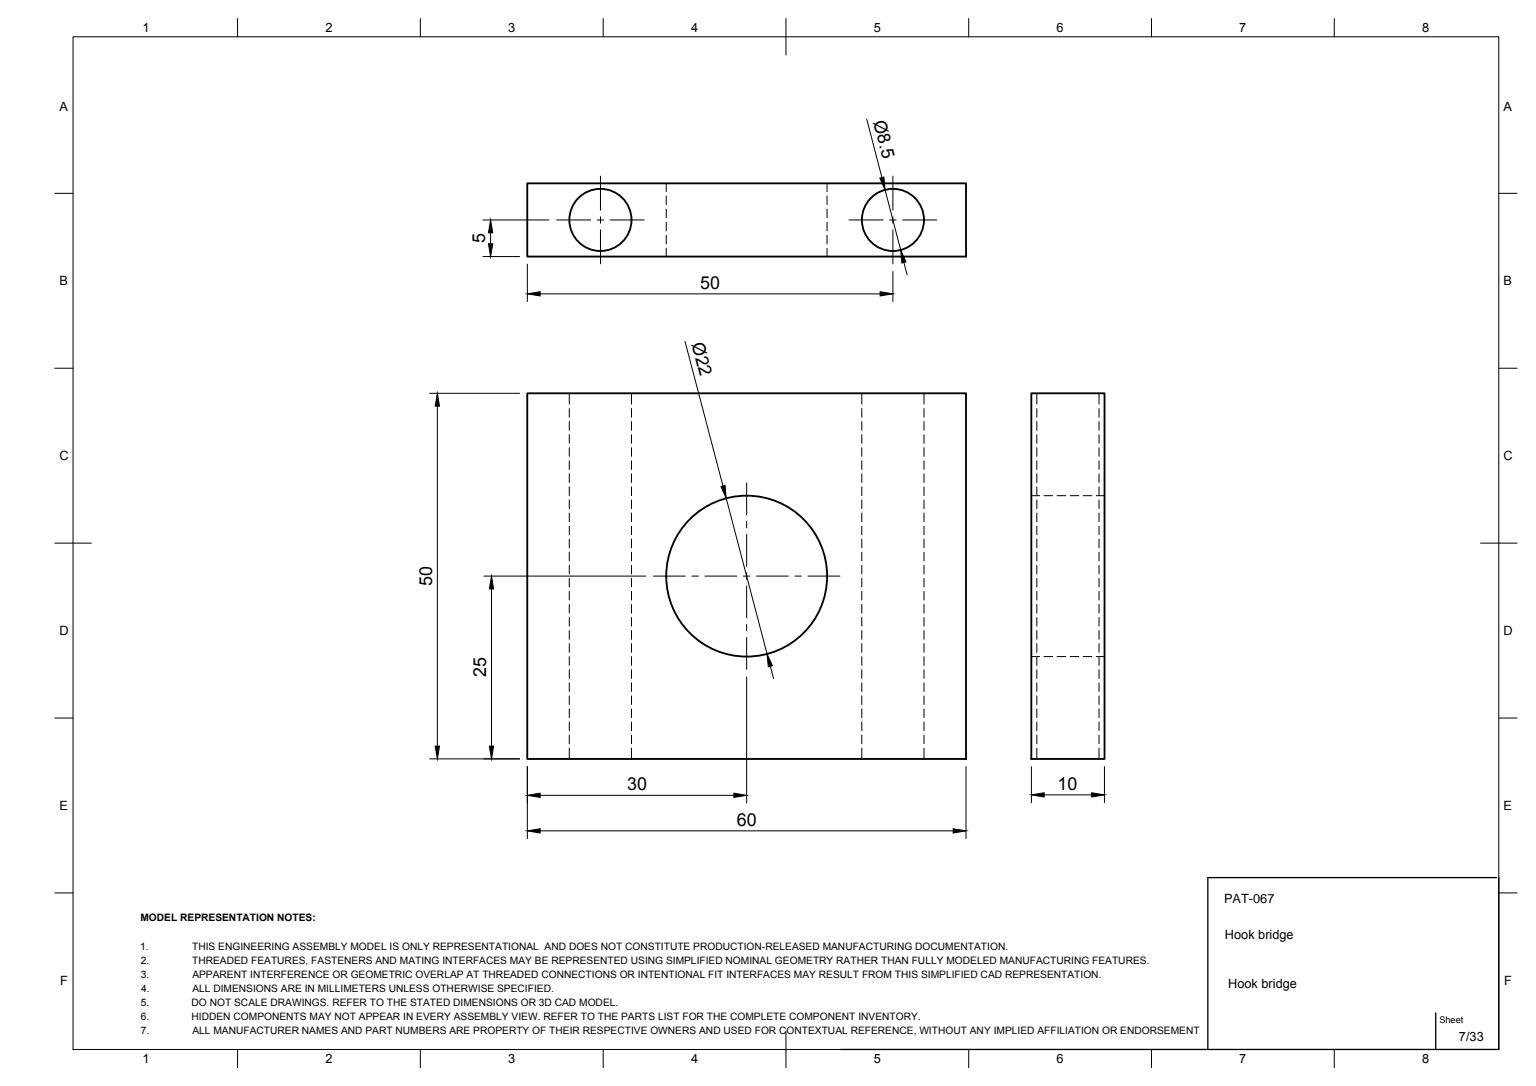
ISO-10303-21;
HEADER;
/* Generated by software containing ST-Developer
 * from STEP Tools, Inc. (www.steptools.com) 
 */

FILE_DESCRIPTION(
/* description */ ('Lifting hook block with sheave'),
/* implementation_level */ '2;1');

FILE_NAME(
/* name */ 'Hook bridge.step',
/* time_stamp */ '2026-10-28T03:23:54-07:00',
/* author */ (''),
/* organization */ (''),
/* preprocessor_version */ 'ST-DEVELOPER v20.2',
/* originating_system */ 'Autodesk Translation Framework v15.17.0.0',
/* authorisation */ '');

FILE_SCHEMA (('AUTOMOTIVE_DESIGN { 1 0 10303 214 3 1 1 }'));
ENDSEC;

DATA;
#10=MECHANICAL_DESIGN_GEOMETRIC_PRESENTATION_REPRESENTATION('',(#353),#9391);
#293=SHAPE_REPRESENTATION_RELATIONSHIP('SRR','None',#9524,#323);
#323=ADVANCED_BREP_SHAPE_REPRESENTATION('',(#391),#9359);
#353=STYLED_ITEM('',(#9773),#391);
#391=MANIFOLD_SOLID_BREP('Body1',#4889);
#506=LINE('',#7866,#794);
#507=LINE('',#7872,#795);
#508=LINE('',#7878,#796);
#509=LINE('',#7883,#797);
#510=LINE('',#7885,#798);
#511=LINE('',#7887,#799);
#512=LINE('',#7888,#800);
#513=LINE('',#7891,#801);
#514=LINE('',#7893,#802);
#515=LINE('',#7894,#803);
#516=LINE('',#7897,#804);
#517=LINE('',#7899,#805);
#518=LINE('',#7900,#806);
#519=LINE('',#7902,#807);
#520=LINE('',#7903,#808);
#794=VECTOR('',#6261,1.1);
#795=VECTOR('',#6268,0.425);
#796=VECTOR('',#6275,0.425);
#797=VECTOR('',#6280,1.);
#798=VECTOR('',#6281,1.);
#799=VECTOR('',#6282,1.);
#800=VECTOR('',#6283,1.);
#801=VECTOR('',#6286,1.);
#802=VECTOR('',#6287,1.);
#803=VECTOR('',#6288,1.);
#804=VECTOR('',#6291,1.);
#805=VECTOR('',#6292,1.);
#806=VECTOR('',#6293,1.);
#807=VECTOR('',#6296,1.);
#808=VECTOR('',#6297,1.);
#1026=CYLINDRICAL_SURFACE('',#5382,1.1);
#1027=CYLINDRICAL_SURFACE('',#5385,0.425);
#1028=CYLINDRICAL_SURFACE('',#5388,0.425);
#1135=FACE_BOUND('',#1593,.T.);
#1136=FACE_BOUND('',#1594,.T.);
#1137=FACE_BOUND('',#1597,.T.);
#1138=FACE_BOUND('',#1598,.T.);
#1139=FACE_BOUND('',#1601,.T.);
#1140=FACE_BOUND('',#1603,.T.);
#1272=FACE_OUTER_BOUND('',#1589,.T.);
#1273=FACE_OUTER_BOUND('',#1590,.T.);
#1274=FACE_OUTER_BOUND('',#1591,.T.);
#1275=FACE_OUTER_BOUND('',#1592,.T.);
#1276=FACE_OUTER_BOUND('',#1595,.T.);
#1277=FACE_OUTER_BOUND('',#1596,.T.);
#1278=FACE_OUTER_BOUND('',#1599,.T.);
#1279=FACE_OUTER_BOUND('',#1600,.T.);
#1280=FACE_OUTER_BOUND('',#1602,.T.);
#1589=EDGE_LOOP('',(#3530,#3531,#3532,#3533));
#1590=EDGE_LOOP('',(#3534,#3535,#3536,#3537));
#1591=EDGE_LOOP('',(#3538,#3539,#3540,#3541));
#1592=EDGE_LOOP('',(#3542,#3543,#3544,#3545));
#1593=EDGE_LOOP('',(#3546));
#1594=EDGE_LOOP('',(#3547));
#1595=EDGE_LOOP('',(#3548,#3549,#3550,#3551));
#1596=EDGE_LOOP('',(#3552,#3553,#3554,#3555));
#1597=EDGE_LOOP('',(#3556));
#1598=EDGE_LOOP('',(#3557));
#1599=EDGE_LOOP('',(#3558,#3559,#3560,#3561));
#1600=EDGE_LOOP('',(#3562,#3563,#3564,#3565));
#1601=EDGE_LOOP('',(#3566));
#1602=EDGE_LOOP('',(#3567,#3568,#3569,#3570));
#1603=EDGE_LOOP('',(#3571));
#1983=CIRCLE('',#5383,1.1);
#1984=CIRCLE('',#5384,1.1);
#1985=CIRCLE('',#5386,0.425);
#1986=CIRCLE('',#5387,0.425);
#1987=CIRCLE('',#5389,0.425);
#1988=CIRCLE('',#5390,0.425);
#2308=VERTEX_POINT('',#7863);
#2309=VERTEX_POINT('',#7865);
#2310=VERTEX_POINT('',#7869);
#2311=VERTEX_POINT('',#7871);
#2312=VERTEX_POINT('',#7875);
#2313=VERTEX_POINT('',#7877);
#2314=VERTEX_POINT('',#7881);
#2315=VERTEX_POINT('',#7882);
#2316=VERTEX_POINT('',#7884);
#2317=VERTEX_POINT('',#7886);
#2318=VERTEX_POINT('',#7890);
#2319=VERTEX_POINT('',#7892);
#2320=VERTEX_POINT('',#7896);
#2321=VERTEX_POINT('',#7898);
#2769=EDGE_CURVE('',#2308,#2308,#1983,.T.);
#2770=EDGE_CURVE('',#2308,#2309,#506,.T.);
#2771=EDGE_CURVE('',#2309,#2309,#1984,.T.);
#2772=EDGE_CURVE('',#2310,#2310,#1985,.T.);
#2773=EDGE_CURVE('',#2310,#2311,#507,.T.);
#2774=EDGE_CURVE('',#2311,#2311,#1986,.T.);
#2775=EDGE_CURVE('',#2312,#2312,#1987,.T.);
#2776=EDGE_CURVE('',#2312,#2313,#508,.T.);
#2777=EDGE_CURVE('',#2313,#2313,#1988,.T.);
#2778=EDGE_CURVE('',#2314,#2315,#509,.T.);
#2779=EDGE_CURVE('',#2315,#2316,#510,.T.);
#2780=EDGE_CURVE('',#2317,#2316,#511,.T.);
#2781=EDGE_CURVE('',#2314,#2317,#512,.T.);
#2782=EDGE_CURVE('',#2318,#2314,#513,.T.);
#2783=EDGE_CURVE('',#2319,#2317,#514,.T.);
#2784=EDGE_CURVE('',#2318,#2319,#515,.T.);
#2785=EDGE_CURVE('',#2320,#2318,#516,.T.);
#2786=EDGE_CURVE('',#2321,#2319,#517,.T.);
#2787=EDGE_CURVE('',#2320,#2321,#518,.T.);
#2788=EDGE_CURVE('',#2315,#2320,#519,.T.);
#2789=EDGE_CURVE('',#2316,#2321,#520,.T.);
#3530=ORIENTED_EDGE('',*,*,#2769,.F.);
#3531=ORIENTED_EDGE('',*,*,#2770,.T.);
#3532=ORIENTED_EDGE('',*,*,#2771,.F.);
#3533=ORIENTED_EDGE('',*,*,#2770,.F.);
#3534=ORIENTED_EDGE('',*,*,#2772,.F.);
#3535=ORIENTED_EDGE('',*,*,#2773,.T.);
#3536=ORIENTED_EDGE('',*,*,#2774,.F.);
#3537=ORIENTED_EDGE('',*,*,#2773,.F.);
#3538=ORIENTED_EDGE('',*,*,#2775,.F.);
#3539=ORIENTED_EDGE('',*,*,#2776,.T.);
#3540=ORIENTED_EDGE('',*,*,#2777,.F.);
#3541=ORIENTED_EDGE('',*,*,#2776,.F.);
#3542=ORIENTED_EDGE('',*,*,#2778,.T.);
#3543=ORIENTED_EDGE('',*,*,#2779,.T.);
#3544=ORIENTED_EDGE('',*,*,#2780,.F.);
#3545=ORIENTED_EDGE('',*,*,#2781,.F.);
#3546=ORIENTED_EDGE('',*,*,#2774,.T.);
#3547=ORIENTED_EDGE('',*,*,#2777,.T.);
#3548=ORIENTED_EDGE('',*,*,#2782,.T.);
#3549=ORIENTED_EDGE('',*,*,#2781,.T.);
#3550=ORIENTED_EDGE('',*,*,#2783,.F.);
#3551=ORIENTED_EDGE('',*,*,#2784,.F.);
#3552=ORIENTED_EDGE('',*,*,#2785,.T.);
#3553=ORIENTED_EDGE('',*,*,#2784,.T.);
#3554=ORIENTED_EDGE('',*,*,#2786,.F.);
#3555=ORIENTED_EDGE('',*,*,#2787,.F.);
#3556=ORIENTED_EDGE('',*,*,#2772,.T.);
#3557=ORIENTED_EDGE('',*,*,#2775,.T.);
#3558=ORIENTED_EDGE('',*,*,#2788,.T.);
#3559=ORIENTED_EDGE('',*,*,#2787,.T.);
#3560=ORIENTED_EDGE('',*,*,#2789,.F.);
#3561=ORIENTED_EDGE('',*,*,#2779,.F.);
#3562=ORIENTED_EDGE('',*,*,#2789,.T.);
#3563=ORIENTED_EDGE('',*,*,#2786,.T.);
#3564=ORIENTED_EDGE('',*,*,#2783,.T.);
#3565=ORIENTED_EDGE('',*,*,#2780,.T.);
#3566=ORIENTED_EDGE('',*,*,#2771,.T.);
#3567=ORIENTED_EDGE('',*,*,#2788,.F.);
#3568=ORIENTED_EDGE('',*,*,#2778,.F.);
#3569=ORIENTED_EDGE('',*,*,#2782,.F.);
#3570=ORIENTED_EDGE('',*,*,#2785,.F.);
#3571=ORIENTED_EDGE('',*,*,#2769,.T.);
#4476=PLANE('',#5391);
#4477=PLANE('',#5392);
#4478=PLANE('',#5393);
#4479=PLANE('',#5394);
#4480=PLANE('',#5395);
#4481=PLANE('',#5396);
#4648=ADVANCED_FACE('',(#1272),#1026,.F.);
#4649=ADVANCED_FACE('',(#1273),#1027,.F.);
#4650=ADVANCED_FACE('',(#1274),#1028,.F.);
#4651=ADVANCED_FACE('',(#1275,#1135,#1136),#4476,.T.);
#4652=ADVANCED_FACE('',(#1276),#4477,.T.);
#4653=ADVANCED_FACE('',(#1277,#1137,#1138),#4478,.T.);
#4654=ADVANCED_FACE('',(#1278),#4479,.T.);
#4655=ADVANCED_FACE('',(#1279,#1139),#4480,.T.);
#4656=ADVANCED_FACE('',(#1280,#1140),#4481,.F.);
#4889=CLOSED_SHELL('',(#4648,#4649,#4650,#4651,#4652,#4653,#4654,#4655,
#4656));
#5381=AXIS2_PLACEMENT_3D('',#7861,#6255,#6256);
#5382=AXIS2_PLACEMENT_3D('',#7862,#6257,#6258);
#5383=AXIS2_PLACEMENT_3D('',#7864,#6259,#6260);
#5384=AXIS2_PLACEMENT_3D('',#7867,#6262,#6263);
#5385=AXIS2_PLACEMENT_3D('',#7868,#6264,#6265);
#5386=AXIS2_PLACEMENT_3D('',#7870,#6266,#6267);
#5387=AXIS2_PLACEMENT_3D('',#7873,#6269,#6270);
#5388=AXIS2_PLACEMENT_3D('',#7874,#6271,#6272);
#5389=AXIS2_PLACEMENT_3D('',#7876,#6273,#6274);
#5390=AXIS2_PLACEMENT_3D('',#7879,#6276,#6277);
#5391=AXIS2_PLACEMENT_3D('',#7880,#6278,#6279);
#5392=AXIS2_PLACEMENT_3D('',#7889,#6284,#6285);
#5393=AXIS2_PLACEMENT_3D('',#7895,#6289,#6290);
#5394=AXIS2_PLACEMENT_3D('',#7901,#6294,#6295);
#5395=AXIS2_PLACEMENT_3D('',#7904,#6298,#6299);
#5396=AXIS2_PLACEMENT_3D('',#7905,#6300,#6301);
#6255=DIRECTION('axis',(0.,0.,1.));
#6256=DIRECTION('refdir',(1.,0.,0.));
#6257=DIRECTION('center_axis',(0.,0.,1.));
#6258=DIRECTION('ref_axis',(1.,0.,0.));
#6259=DIRECTION('center_axis',(0.,0.,1.));
#6260=DIRECTION('ref_axis',(1.,0.,0.));
#6261=DIRECTION('',(0.,0.,1.));
#6262=DIRECTION('center_axis',(0.,0.,-1.));
#6263=DIRECTION('ref_axis',(1.,0.,0.));
#6264=DIRECTION('center_axis',(0.,1.,0.));
#6265=DIRECTION('ref_axis',(1.,0.,0.));
#6266=DIRECTION('center_axis',(0.,1.,0.));
#6267=DIRECTION('ref_axis',(1.,0.,0.));
#6268=DIRECTION('',(0.,1.,0.));
#6269=DIRECTION('center_axis',(0.,-1.,0.));
#6270=DIRECTION('ref_axis',(1.,0.,0.));
#6271=DIRECTION('center_axis',(0.,1.,0.));
#6272=DIRECTION('ref_axis',(1.,0.,0.));
#6273=DIRECTION('center_axis',(0.,1.,0.));
#6274=DIRECTION('ref_axis',(1.,0.,0.));
#6275=DIRECTION('',(0.,1.,0.));
#6276=DIRECTION('center_axis',(0.,-1.,0.));
#6277=DIRECTION('ref_axis',(1.,0.,0.));
#6278=DIRECTION('center_axis',(0.,1.,0.));
#6279=DIRECTION('ref_axis',(-1.,0.,0.));
#6280=DIRECTION('',(-1.,0.,0.));
#6281=DIRECTION('',(0.,0.,1.));
#6282=DIRECTION('',(-1.,0.,0.));
#6283=DIRECTION('',(0.,0.,1.));
#6284=DIRECTION('center_axis',(1.,0.,0.));
#6285=DIRECTION('ref_axis',(0.,1.,0.));
#6286=DIRECTION('',(0.,1.,0.));
#6287=DIRECTION('',(0.,1.,0.));
#6288=DIRECTION('',(0.,0.,1.));
#6289=DIRECTION('center_axis',(0.,-1.,0.));
#6290=DIRECTION('ref_axis',(1.,0.,0.));
#6291=DIRECTION('',(1.,0.,0.));
#6292=DIRECTION('',(1.,0.,0.));
#6293=DIRECTION('',(0.,0.,1.));
#6294=DIRECTION('center_axis',(-1.,0.,0.));
#6295=DIRECTION('ref_axis',(0.,-1.,0.));
#6296=DIRECTION('',(0.,-1.,0.));
#6297=DIRECTION('',(0.,-1.,0.));
#6298=DIRECTION('center_axis',(0.,0.,1.));
#6299=DIRECTION('ref_axis',(1.,0.,0.));
#6300=DIRECTION('center_axis',(0.,0.,1.));
#6301=DIRECTION('ref_axis',(1.,0.,0.));
#7861=CARTESIAN_POINT('',(0.,0.,0.));
#7862=CARTESIAN_POINT('Origin',(0.,0.,4.4));
#7863=CARTESIAN_POINT('',(-1.1,-1.34711147906209E-16,4.5));
#7864=CARTESIAN_POINT('Origin',(0.,0.,4.5));
#7865=CARTESIAN_POINT('',(-1.1,1.34711147906209E-16,5.5));
#7866=CARTESIAN_POINT('',(-1.1,-1.34711147906209E-16,4.4));
#7867=CARTESIAN_POINT('Origin',(0.,0.,5.5));
#7868=CARTESIAN_POINT('Origin',(-2.,-2.6,5.));
#7869=CARTESIAN_POINT('',(-2.425,-2.5,5.));
#7870=CARTESIAN_POINT('Origin',(-2.,-2.5,5.));
#7871=CARTESIAN_POINT('',(-2.425,2.5,5.));
#7872=CARTESIAN_POINT('',(-2.425,-2.6,5.));
#7873=CARTESIAN_POINT('Origin',(-2.,2.5,5.));
#7874=CARTESIAN_POINT('Origin',(2.,-2.6,5.));
#7875=CARTESIAN_POINT('',(1.575,-2.5,5.));
#7876=CARTESIAN_POINT('Origin',(2.,-2.5,5.));
#7877=CARTESIAN_POINT('',(1.575,2.5,5.));
#7878=CARTESIAN_POINT('',(1.575,-2.6,5.));
#7879=CARTESIAN_POINT('Origin',(2.,2.5,5.));
#7880=CARTESIAN_POINT('Origin',(3.,2.5,4.5));
#7881=CARTESIAN_POINT('',(3.,2.5,4.5));
#7882=CARTESIAN_POINT('',(-3.,2.5,4.5));
#7883=CARTESIAN_POINT('',(3.,2.5,4.5));
#7884=CARTESIAN_POINT('',(-3.,2.5,5.5));
#7885=CARTESIAN_POINT('',(-3.,2.5,4.5));
#7886=CARTESIAN_POINT('',(3.,2.5,5.5));
#7887=CARTESIAN_POINT('',(3.,2.5,5.5));
#7888=CARTESIAN_POINT('',(3.,2.5,4.5));
#7889=CARTESIAN_POINT('Origin',(3.,-2.5,4.5));
#7890=CARTESIAN_POINT('',(3.,-2.5,4.5));
#7891=CARTESIAN_POINT('',(3.,-2.5,4.5));
#7892=CARTESIAN_POINT('',(3.,-2.5,5.5));
#7893=CARTESIAN_POINT('',(3.,-2.5,5.5));
#7894=CARTESIAN_POINT('',(3.,-2.5,4.5));
#7895=CARTESIAN_POINT('Origin',(-3.,-2.5,4.5));
#7896=CARTESIAN_POINT('',(-3.,-2.5,4.5));
#7897=CARTESIAN_POINT('',(-3.,-2.5,4.5));
#7898=CARTESIAN_POINT('',(-3.,-2.5,5.5));
#7899=CARTESIAN_POINT('',(-3.,-2.5,5.5));
#7900=CARTESIAN_POINT('',(-3.,-2.5,4.5));
#7901=CARTESIAN_POINT('Origin',(-3.,2.5,4.5));
#7902=CARTESIAN_POINT('',(-3.,2.5,4.5));
#7903=CARTESIAN_POINT('',(-3.,2.5,5.5));
#7904=CARTESIAN_POINT('Origin',(0.,0.,5.5));
#7905=CARTESIAN_POINT('Origin',(0.,0.,4.5));
#9322=UNCERTAINTY_MEASURE_WITH_UNIT(LENGTH_MEASURE(0.001),#9392,
'DISTANCE_ACCURACY_VALUE',
'Maximum model space distance between geometric entities at asserted c
onnectivities');
#9354=UNCERTAINTY_MEASURE_WITH_UNIT(LENGTH_MEASURE(0.001),#9392,
'DISTANCE_ACCURACY_VALUE',
'Maximum model space distance between geometric entities at asserted c
onnectivities');
#9359=(
GEOMETRIC_REPRESENTATION_CONTEXT(3)
GLOBAL_UNCERTAINTY_ASSIGNED_CONTEXT((#9322))
GLOBAL_UNIT_ASSIGNED_CONTEXT((#9392,#9394,#9395))
REPRESENTATION_CONTEXT('','3D')
);
#9391=(
GEOMETRIC_REPRESENTATION_CONTEXT(3)
GLOBAL_UNCERTAINTY_ASSIGNED_CONTEXT((#9354))
GLOBAL_UNIT_ASSIGNED_CONTEXT((#9392,#9394,#9395))
REPRESENTATION_CONTEXT('','3D')
);
#9392=(
LENGTH_UNIT()
NAMED_UNIT(*)
SI_UNIT(.CENTI.,.METRE.)
);
#9394=(
NAMED_UNIT(*)
PLANE_ANGLE_UNIT()
SI_UNIT($,.RADIAN.)
);
#9395=(
NAMED_UNIT(*)
SI_UNIT($,.STERADIAN.)
SOLID_ANGLE_UNIT()
);
#9400=SHAPE_DEFINITION_REPRESENTATION(#9436,#9524);
#9436=PRODUCT_DEFINITION_SHAPE('',$,#9561);
#9524=SHAPE_REPRESENTATION('',(#5381),#9359);
#9556=PRODUCT_DEFINITION_CONTEXT('part definition',#9666,'design');
#9561=PRODUCT_DEFINITION('Hook bridge','Hook bridge',#9597,#9556);
#9597=PRODUCT_DEFINITION_FORMATION('',$,#9672);
#9666=APPLICATION_CONTEXT(
'Core Data for Automotive Mechanical Design Process');
#9667=PRODUCT_CONTEXT('part definition',#9666,'mechanical');
#9672=PRODUCT('Hook bridge','Hook bridge','Hook bridge',(#9667));
#9767=COLOUR_RGB('Off White',0.89,0.88,0.83);
#9768=FILL_AREA_STYLE_COLOUR('',#9767);
#9769=FILL_AREA_STYLE('',(#9768));
#9770=SURFACE_STYLE_FILL_AREA(#9769);
#9771=SURFACE_SIDE_STYLE('',(#9770));
#9772=SURFACE_STYLE_USAGE(.BOTH.,#9771);
#9773=PRESENTATION_STYLE_ASSIGNMENT((#9772));
ENDSEC;
END-ISO-10303-21;
